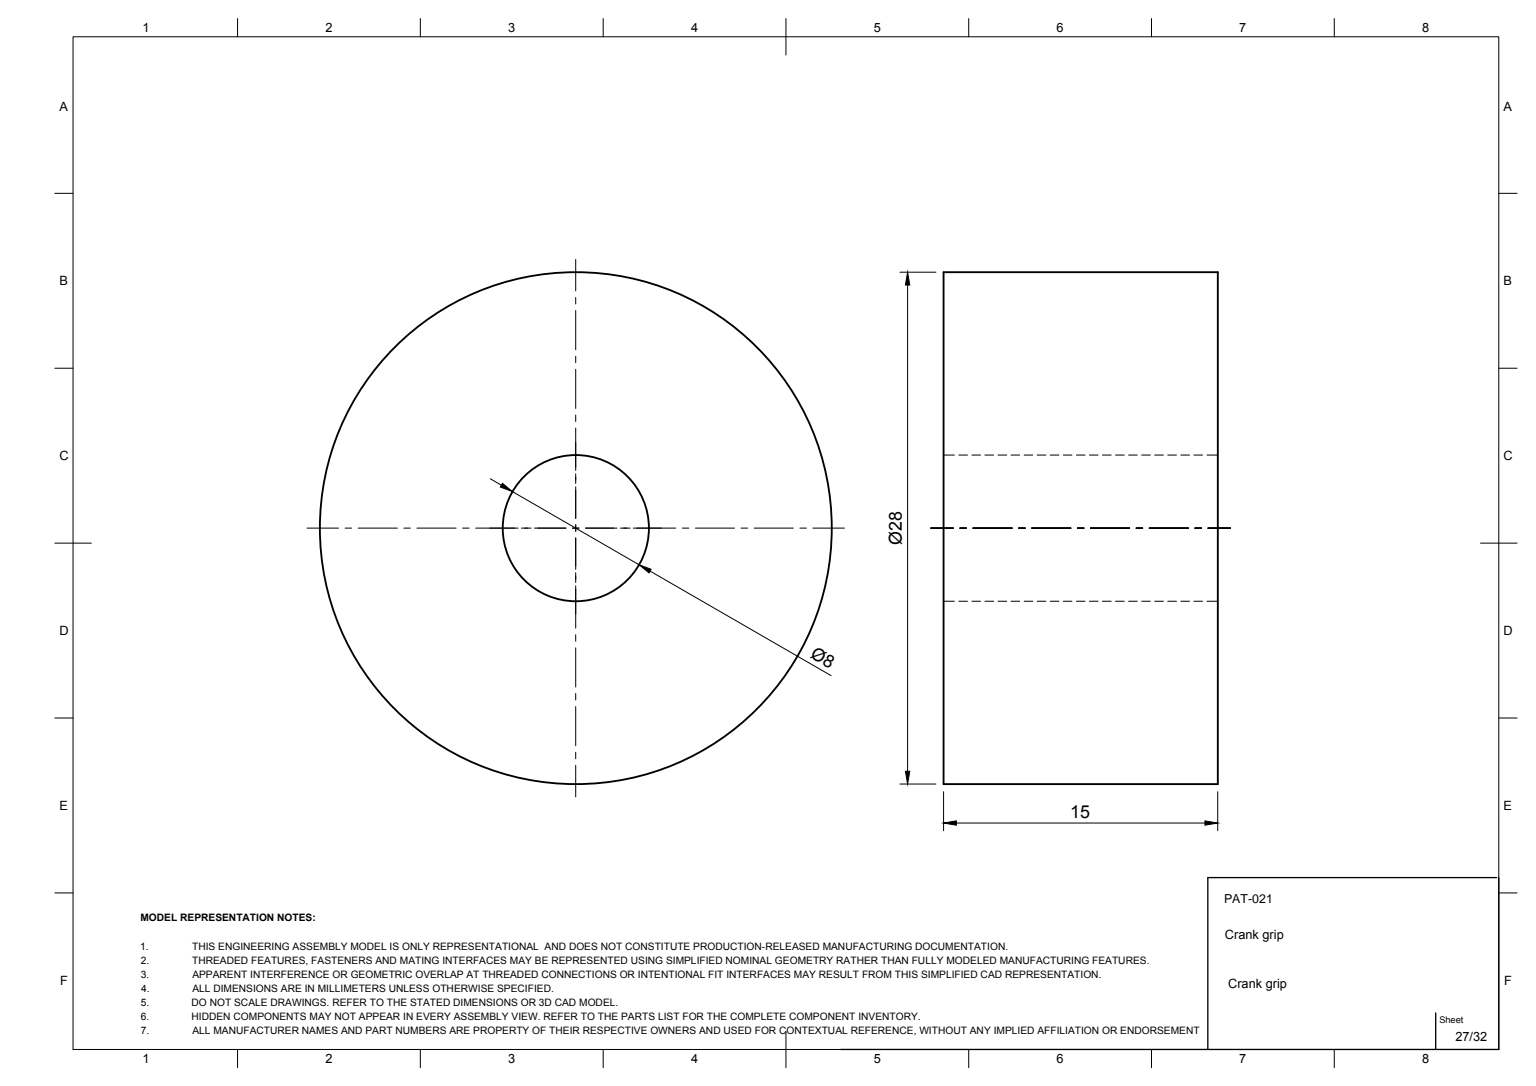
ISO-10303-21;
HEADER;
/* Generated by software containing ST-Developer
 * from STEP Tools, Inc. (www.steptools.com) 
 */

FILE_DESCRIPTION(
/* description */ ('Chain-less indexing wheel (Geneva) drive'),
/* implementation_level */ '2;1');

FILE_NAME(
/* name */ 'Crank grip.step',
/* time_stamp */ '2026-10-28T03:25:22-07:00',
/* author */ (''),
/* organization */ (''),
/* preprocessor_version */ 'ST-DEVELOPER v20.2',
/* originating_system */ 'Autodesk Translation Framework v15.17.0.0',
/* authorisation */ '');

FILE_SCHEMA (('AUTOMOTIVE_DESIGN { 1 0 10303 214 3 1 1 }'));
ENDSEC;

DATA;
#10=MECHANICAL_DESIGN_GEOMETRIC_PRESENTATION_REPRESENTATION('',(#330),#10957);
#272=SHAPE_REPRESENTATION_RELATIONSHIP('SRR','None',#11087,#297);
#297=ADVANCED_BREP_SHAPE_REPRESENTATION('',(#362),#10950);
#330=STYLED_ITEM('',(#11294),#362);
#362=MANIFOLD_SOLID_BREP('Body1',#5727);
#453=FACE_BOUND('',#1305,.T.);
#454=FACE_BOUND('',#1307,.T.);
#587=PLANE('',#6523);
#588=PLANE('',#6524);
#883=FACE_OUTER_BOUND('',#1302,.T.);
#884=FACE_OUTER_BOUND('',#1303,.T.);
#885=FACE_OUTER_BOUND('',#1304,.T.);
#886=FACE_OUTER_BOUND('',#1306,.T.);
#1302=EDGE_LOOP('',(#4731,#4732,#4733,#4734));
#1303=EDGE_LOOP('',(#4735,#4736,#4737,#4738));
#1304=EDGE_LOOP('',(#4739));
#1305=EDGE_LOOP('',(#4740));
#1306=EDGE_LOOP('',(#4741));
#1307=EDGE_LOOP('',(#4742));
#1638=LINE('',#10208,#2012);
#1639=LINE('',#10214,#2013);
#2012=VECTOR('',#7982,0.4);
#2013=VECTOR('',#7989,1.4);
#2418=CIRCLE('',#6518,0.4);
#2419=CIRCLE('',#6519,0.4);
#2420=CIRCLE('',#6521,1.4);
#2421=CIRCLE('',#6522,1.4);
#2830=VERTEX_POINT('',#10205);
#2831=VERTEX_POINT('',#10207);
#2832=VERTEX_POINT('',#10211);
#2833=VERTEX_POINT('',#10213);
#3491=EDGE_CURVE('',#2830,#2830,#2418,.T.);
#3492=EDGE_CURVE('',#2830,#2831,#1638,.T.);
#3493=EDGE_CURVE('',#2831,#2831,#2419,.T.);
#3494=EDGE_CURVE('',#2832,#2832,#2420,.T.);
#3495=EDGE_CURVE('',#2832,#2833,#1639,.T.);
#3496=EDGE_CURVE('',#2833,#2833,#2421,.T.);
#4731=ORIENTED_EDGE('',*,*,#3491,.F.);
#4732=ORIENTED_EDGE('',*,*,#3492,.T.);
#4733=ORIENTED_EDGE('',*,*,#3493,.T.);
#4734=ORIENTED_EDGE('',*,*,#3492,.F.);
#4735=ORIENTED_EDGE('',*,*,#3494,.F.);
#4736=ORIENTED_EDGE('',*,*,#3495,.T.);
#4737=ORIENTED_EDGE('',*,*,#3496,.T.);
#4738=ORIENTED_EDGE('',*,*,#3495,.F.);
#4739=ORIENTED_EDGE('',*,*,#3494,.T.);
#4740=ORIENTED_EDGE('',*,*,#3491,.T.);
#4741=ORIENTED_EDGE('',*,*,#3496,.F.);
#4742=ORIENTED_EDGE('',*,*,#3493,.F.);
#5333=CYLINDRICAL_SURFACE('',#6517,0.4);
#5334=CYLINDRICAL_SURFACE('',#6520,1.4);
#5597=ADVANCED_FACE('',(#883),#5333,.F.);
#5598=ADVANCED_FACE('',(#884),#5334,.T.);
#5599=ADVANCED_FACE('',(#885,#453),#587,.T.);
#5600=ADVANCED_FACE('',(#886,#454),#588,.F.);
#5727=CLOSED_SHELL('',(#5597,#5598,#5599,#5600));
#6516=AXIS2_PLACEMENT_3D('',#10203,#7976,#7977);
#6517=AXIS2_PLACEMENT_3D('',#10204,#7978,#7979);
#6518=AXIS2_PLACEMENT_3D('',#10206,#7980,#7981);
#6519=AXIS2_PLACEMENT_3D('',#10209,#7983,#7984);
#6520=AXIS2_PLACEMENT_3D('',#10210,#7985,#7986);
#6521=AXIS2_PLACEMENT_3D('',#10212,#7987,#7988);
#6522=AXIS2_PLACEMENT_3D('',#10215,#7990,#7991);
#6523=AXIS2_PLACEMENT_3D('',#10216,#7992,#7993);
#6524=AXIS2_PLACEMENT_3D('',#10217,#7994,#7995);
#7976=DIRECTION('axis',(0.,0.,1.));
#7977=DIRECTION('refdir',(1.,0.,0.));
#7978=DIRECTION('center_axis',(0.,0.,1.));
#7979=DIRECTION('ref_axis',(1.,0.,0.));
#7980=DIRECTION('center_axis',(0.,0.,-1.));
#7981=DIRECTION('ref_axis',(1.,0.,0.));
#7982=DIRECTION('',(0.,0.,-1.));
#7983=DIRECTION('center_axis',(0.,0.,-1.));
#7984=DIRECTION('ref_axis',(1.,0.,0.));
#7985=DIRECTION('center_axis',(0.,0.,1.));
#7986=DIRECTION('ref_axis',(1.,0.,0.));
#7987=DIRECTION('center_axis',(0.,0.,1.));
#7988=DIRECTION('ref_axis',(1.,0.,0.));
#7989=DIRECTION('',(0.,0.,-1.));
#7990=DIRECTION('center_axis',(0.,0.,1.));
#7991=DIRECTION('ref_axis',(1.,0.,0.));
#7992=DIRECTION('center_axis',(0.,0.,1.));
#7993=DIRECTION('ref_axis',(1.,0.,0.));
#7994=DIRECTION('center_axis',(0.,0.,1.));
#7995=DIRECTION('ref_axis',(1.,0.,0.));
#10203=CARTESIAN_POINT('',(0.,0.,0.));
#10204=CARTESIAN_POINT('Origin',(0.,0.,7.));
#10205=CARTESIAN_POINT('',(-0.4,-4.89858719658941E-17,8.5));
#10206=CARTESIAN_POINT('Origin',(0.,0.,8.5));
#10207=CARTESIAN_POINT('',(-0.4,-4.89858719658941E-17,7.));
#10208=CARTESIAN_POINT('',(-0.4,-4.89858719658941E-17,7.));
#10209=CARTESIAN_POINT('Origin',(0.,0.,7.));
#10210=CARTESIAN_POINT('Origin',(0.,0.,7.));
#10211=CARTESIAN_POINT('',(-1.4,-1.71450551880629E-16,8.5));
#10212=CARTESIAN_POINT('Origin',(0.,0.,8.5));
#10213=CARTESIAN_POINT('',(-1.4,-1.71450551880629E-16,7.));
#10214=CARTESIAN_POINT('',(-1.4,-1.71450551880629E-16,7.));
#10215=CARTESIAN_POINT('Origin',(0.,0.,7.));
#10216=CARTESIAN_POINT('Origin',(0.,0.,8.5));
#10217=CARTESIAN_POINT('Origin',(0.,0.,7.));
#10919=UNCERTAINTY_MEASURE_WITH_UNIT(LENGTH_MEASURE(0.001),#10958,
'DISTANCE_ACCURACY_VALUE',
'Maximum model space distance between geometric entities at asserted c
onnectivities');
#10926=UNCERTAINTY_MEASURE_WITH_UNIT(LENGTH_MEASURE(0.001),#10958,
'DISTANCE_ACCURACY_VALUE',
'Maximum model space distance between geometric entities at asserted c
onnectivities');
#10950=(
GEOMETRIC_REPRESENTATION_CONTEXT(3)
GLOBAL_UNCERTAINTY_ASSIGNED_CONTEXT((#10919))
GLOBAL_UNIT_ASSIGNED_CONTEXT((#10958,#10960,#10961))
REPRESENTATION_CONTEXT('','3D')
);
#10957=(
GEOMETRIC_REPRESENTATION_CONTEXT(3)
GLOBAL_UNCERTAINTY_ASSIGNED_CONTEXT((#10926))
GLOBAL_UNIT_ASSIGNED_CONTEXT((#10958,#10960,#10961))
REPRESENTATION_CONTEXT('','3D')
);
#10958=(
LENGTH_UNIT()
NAMED_UNIT(*)
SI_UNIT(.CENTI.,.METRE.)
);
#10960=(
NAMED_UNIT(*)
PLANE_ANGLE_UNIT()
SI_UNIT($,.RADIAN.)
);
#10961=(
NAMED_UNIT(*)
SI_UNIT($,.STERADIAN.)
SOLID_ANGLE_UNIT()
);
#10985=SHAPE_DEFINITION_REPRESENTATION(#11020,#11087);
#11020=PRODUCT_DEFINITION_SHAPE('',$,#11118);
#11087=SHAPE_REPRESENTATION('',(#6516),#10950);
#11094=PRODUCT_DEFINITION_CONTEXT('part definition',#11186,'design');
#11118=PRODUCT_DEFINITION('Crank grip','Crank grip',#11148,#11094);
#11148=PRODUCT_DEFINITION_FORMATION('',$,#11211);
#11186=APPLICATION_CONTEXT(
'Core Data for Automotive Mechanical Design Process');
#11187=PRODUCT_CONTEXT('part definition',#11186,'mechanical');
#11211=PRODUCT('Crank grip','Crank grip','Crank grip',(#11187));
#11288=COLOUR_RGB('Black',0.12,0.14,0.17);
#11289=FILL_AREA_STYLE_COLOUR('',#11288);
#11290=FILL_AREA_STYLE('',(#11289));
#11291=SURFACE_STYLE_FILL_AREA(#11290);
#11292=SURFACE_SIDE_STYLE('',(#11291));
#11293=SURFACE_STYLE_USAGE(.BOTH.,#11292);
#11294=PRESENTATION_STYLE_ASSIGNMENT((#11293));
ENDSEC;
END-ISO-10303-21;
